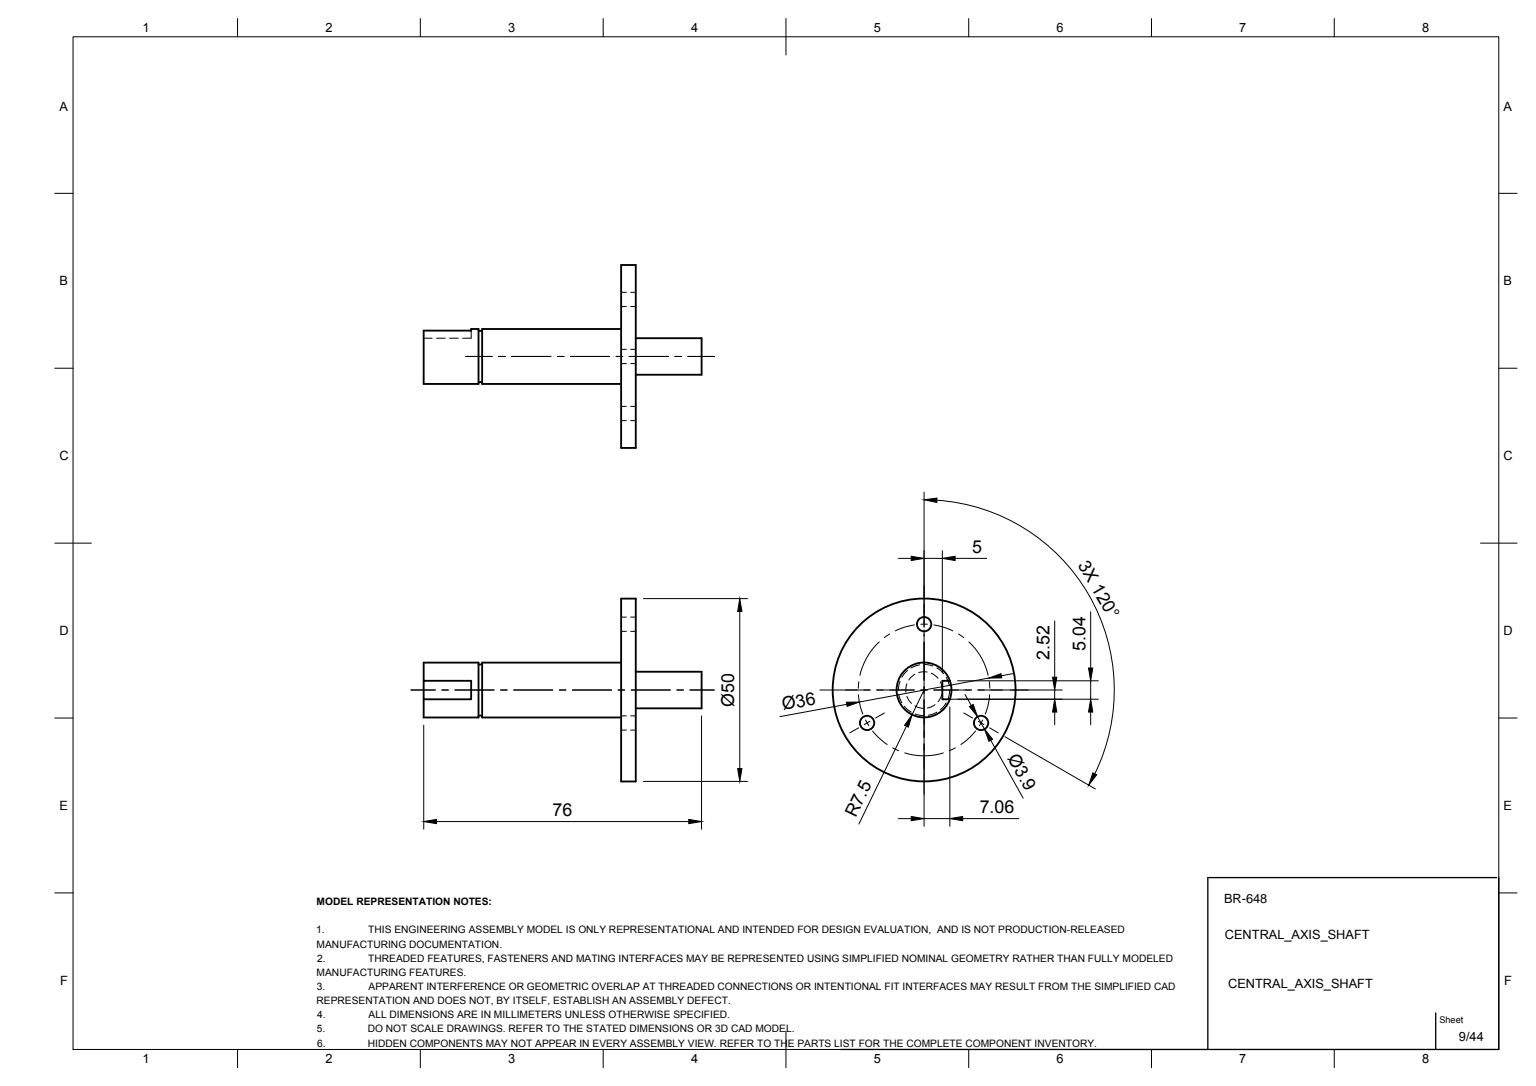
ISO-10303-21;
HEADER;
FILE_DESCRIPTION((''),'2;1');
FILE_NAME('CENTRAL_AXIS_SHAFT.step','2026-10-01T22:05:39-07:00',(''),(''),'','','');
FILE_SCHEMA (('AUTOMOTIVE_DESIGN { 1 0 10303 214 3 1 1 }'));
ENDSEC;
DATA;
#10=MECHANICAL_DESIGN_GEOMETRIC_PRESENTATION_REPRESENTATION('',(#609),#24628);
#525=SHAPE_REPRESENTATION_RELATIONSHIP('SRR','None',#24797,#567) ;
#567=ADVANCED_BREP_SHAPE_REPRESENTATION('',(#651),#24587) ;
#609=STYLED_ITEM('',(#25030),#651) ;
#651=MANIFOLD_SOLID_BREP('CENTRAL_AXIS_SHAFT',#13118) ;
#749=FACE_BOUND('',#3864,.T.) ;
#750=FACE_BOUND('',#3866,.T.) ;
#751=FACE_BOUND('',#3872,.T.) ;
#752=FACE_BOUND('',#3873,.T.) ;
#753=FACE_BOUND('',#3874,.T.) ;
#754=FACE_BOUND('',#3875,.T.) ;
#755=FACE_BOUND('',#3881,.T.) ;
#756=FACE_BOUND('',#3882,.T.) ;
#757=FACE_BOUND('',#3883,.T.) ;
#758=FACE_BOUND('',#3884,.T.) ;
#1071=LINE('',#20189,#1907) ;
#1072=LINE('',#20191,#1908) ;
#1073=LINE('',#20193,#1909) ;
#1074=LINE('',#20194,#1910) ;
#1075=LINE('',#20199,#1911) ;
#1076=LINE('',#20200,#1912) ;
#1077=LINE('',#20204,#1913) ;
#1078=LINE('',#20205,#1914) ;
#1079=LINE('',#20206,#1915) ;
#1080=LINE('',#20208,#1916) ;
#1081=LINE('',#20213,#1917) ;
#1082=LINE('',#20220,#1918) ;
#1083=LINE('',#20229,#1919) ;
#1084=LINE('',#20234,#1920) ;
#1085=LINE('',#20240,#1921) ;
#1086=LINE('',#20246,#1922) ;
#1087=LINE('',#20254,#1923) ;
#1088=LINE('',#20259,#1924) ;
#1907=VECTOR('',#15836,1.) ;
#1908=VECTOR('',#15837,1.) ;
#1909=VECTOR('',#15838,1.) ;
#1910=VECTOR('',#15839,1.) ;
#1911=VECTOR('',#15844,1.) ;
#1912=VECTOR('',#15845,1.) ;
#1913=VECTOR('',#15848,1.) ;
#1914=VECTOR('',#15849,1.) ;
#1915=VECTOR('',#15850,1.) ;
#1916=VECTOR('',#15853,1.) ;
#1917=VECTOR('',#15858,0.75) ;
#1918=VECTOR('',#15867,0.7) ;
#1919=VECTOR('',#15880,0.75) ;
#1920=VECTOR('',#15885,0.195) ;
#1921=VECTOR('',#15892,0.195) ;
#1922=VECTOR('',#15899,0.195) ;
#1923=VECTOR('',#15910,2.5) ;
#1924=VECTOR('',#15915,0.5) ;
#2717=CYLINDRICAL_SURFACE('',#13844,0.75) ;
#2718=CYLINDRICAL_SURFACE('',#13848,0.7) ;
#2719=CYLINDRICAL_SURFACE('',#13854,0.75) ;
#2720=CYLINDRICAL_SURFACE('',#13856,0.195) ;
#2721=CYLINDRICAL_SURFACE('',#13859,0.195) ;
#2722=CYLINDRICAL_SURFACE('',#13862,0.195) ;
#2723=CYLINDRICAL_SURFACE('',#13867,2.5) ;
#2724=CYLINDRICAL_SURFACE('',#13869,0.5) ;
#3027=FACE_OUTER_BOUND('',#3857,.T.) ;
#3028=FACE_OUTER_BOUND('',#3858,.T.) ;
#3029=FACE_OUTER_BOUND('',#3859,.T.) ;
#3030=FACE_OUTER_BOUND('',#3860,.T.) ;
#3031=FACE_OUTER_BOUND('',#3861,.T.) ;
#3032=FACE_OUTER_BOUND('',#3862,.T.) ;
#3033=FACE_OUTER_BOUND('',#3863,.T.) ;
#3034=FACE_OUTER_BOUND('',#3865,.T.) ;
#3035=FACE_OUTER_BOUND('',#3867,.T.) ;
#3036=FACE_OUTER_BOUND('',#3868,.T.) ;
#3037=FACE_OUTER_BOUND('',#3869,.T.) ;
#3038=FACE_OUTER_BOUND('',#3870,.T.) ;
#3039=FACE_OUTER_BOUND('',#3871,.T.) ;
#3040=FACE_OUTER_BOUND('',#3876,.T.) ;
#3041=FACE_OUTER_BOUND('',#3877,.T.) ;
#3042=FACE_OUTER_BOUND('',#3878,.T.) ;
#3043=FACE_OUTER_BOUND('',#3879,.T.) ;
#3044=FACE_OUTER_BOUND('',#3880,.T.) ;
#3857=EDGE_LOOP('',(#8847,#8848,#8849,#8850)) ;
#3858=EDGE_LOOP('',(#8851,#8852,#8853,#8854)) ;
#3859=EDGE_LOOP('',(#8855,#8856,#8857,#8858)) ;
#3860=EDGE_LOOP('',(#8859,#8860,#8861,#8862)) ;
#3861=EDGE_LOOP('',(#8863,#8864,#8865,#8866,#8867,#8868,#8869,#8870)) ;
#3862=EDGE_LOOP('',(#8871,#8872,#8873,#8874)) ;
#3863=EDGE_LOOP('',(#8875)) ;
#3864=EDGE_LOOP('',(#8876)) ;
#3865=EDGE_LOOP('',(#8877)) ;
#3866=EDGE_LOOP('',(#8878)) ;
#3867=EDGE_LOOP('',(#8879,#8880,#8881,#8882)) ;
#3868=EDGE_LOOP('',(#8883,#8884,#8885,#8886)) ;
#3869=EDGE_LOOP('',(#8887,#8888,#8889,#8890)) ;
#3870=EDGE_LOOP('',(#8891,#8892,#8893,#8894)) ;
#3871=EDGE_LOOP('',(#8895)) ;
#3872=EDGE_LOOP('',(#8896)) ;
#3873=EDGE_LOOP('',(#8897)) ;
#3874=EDGE_LOOP('',(#8898)) ;
#3875=EDGE_LOOP('',(#8899)) ;
#3876=EDGE_LOOP('',(#8900,#8901,#8902,#8903)) ;
#3877=EDGE_LOOP('',(#8904,#8905,#8906,#8907)) ;
#3878=EDGE_LOOP('',(#8908)) ;
#3879=EDGE_LOOP('',(#8909,#8910,#8911,#8912,#8913)) ;
#3880=EDGE_LOOP('',(#8914)) ;
#3881=EDGE_LOOP('',(#8915)) ;
#3882=EDGE_LOOP('',(#8916)) ;
#3883=EDGE_LOOP('',(#8917)) ;
#3884=EDGE_LOOP('',(#8918)) ;
#4856=CIRCLE('',#13841,0.75) ;
#4857=CIRCLE('',#13845,0.75) ;
#4858=CIRCLE('',#13846,0.75) ;
#4859=CIRCLE('',#13847,0.75) ;
#4860=CIRCLE('',#13849,0.7) ;
#4861=CIRCLE('',#13850,0.7) ;
#4862=CIRCLE('',#13853,0.75) ;
#4863=CIRCLE('',#13855,0.75) ;
#4864=CIRCLE('',#13857,0.195) ;
#4865=CIRCLE('',#13858,0.195) ;
#4866=CIRCLE('',#13860,0.195) ;
#4867=CIRCLE('',#13861,0.195) ;
#4868=CIRCLE('',#13863,0.195) ;
#4869=CIRCLE('',#13864,0.195) ;
#4870=CIRCLE('',#13866,2.5) ;
#4871=CIRCLE('',#13868,2.5) ;
#4872=CIRCLE('',#13870,0.5) ;
#4873=CIRCLE('',#13871,0.5) ;
#5657=VERTEX_POINT('',#20187) ;
#5658=VERTEX_POINT('',#20188) ;
#5659=VERTEX_POINT('',#20190) ;
#5660=VERTEX_POINT('',#20192) ;
#5661=VERTEX_POINT('',#20196) ;
#5662=VERTEX_POINT('',#20198) ;
#5663=VERTEX_POINT('',#20202) ;
#5664=VERTEX_POINT('',#20203) ;
#5665=VERTEX_POINT('',#20210) ;
#5666=VERTEX_POINT('',#20212) ;
#5667=VERTEX_POINT('',#20217) ;
#5668=VERTEX_POINT('',#20219) ;
#5669=VERTEX_POINT('',#20224) ;
#5670=VERTEX_POINT('',#20227) ;
#5671=VERTEX_POINT('',#20231) ;
#5672=VERTEX_POINT('',#20233) ;
#5673=VERTEX_POINT('',#20237) ;
#5674=VERTEX_POINT('',#20239) ;
#5675=VERTEX_POINT('',#20243) ;
#5676=VERTEX_POINT('',#20245) ;
#5677=VERTEX_POINT('',#20249) ;
#5678=VERTEX_POINT('',#20252) ;
#5679=VERTEX_POINT('',#20256) ;
#5680=VERTEX_POINT('',#20258) ;
#6913=EDGE_CURVE('',#5657,#5658,#1071,.T.) ;
#6914=EDGE_CURVE('',#5659,#5657,#1072,.T.) ;
#6915=EDGE_CURVE('',#5660,#5659,#1073,.T.) ;
#6916=EDGE_CURVE('',#5658,#5660,#1074,.T.) ;
#6917=EDGE_CURVE('',#5660,#5661,#4856,.T.) ;
#6918=EDGE_CURVE('',#5659,#5662,#1075,.T.) ;
#6919=EDGE_CURVE('',#5662,#5661,#1076,.T.) ;
#6920=EDGE_CURVE('',#5663,#5664,#1077,.T.) ;
#6921=EDGE_CURVE('',#5661,#5663,#1078,.T.) ;
#6922=EDGE_CURVE('',#5664,#5662,#1079,.T.) ;
#6923=EDGE_CURVE('',#5664,#5657,#1080,.T.) ;
#6924=EDGE_CURVE('',#5665,#5665,#4857,.T.) ;
#6925=EDGE_CURVE('',#5665,#5666,#1081,.T.) ;
#6926=EDGE_CURVE('',#5658,#5666,#4858,.T.) ;
#6927=EDGE_CURVE('',#5666,#5663,#4859,.T.) ;
#6928=EDGE_CURVE('',#5667,#5667,#4860,.T.) ;
#6929=EDGE_CURVE('',#5667,#5668,#1082,.T.) ;
#6930=EDGE_CURVE('',#5668,#5668,#4861,.T.) ;
#6931=EDGE_CURVE('',#5669,#5669,#4862,.T.) ;
#6932=EDGE_CURVE('',#5670,#5670,#4863,.T.) ;
#6933=EDGE_CURVE('',#5670,#5669,#1083,.T.) ;
#6934=EDGE_CURVE('',#5671,#5671,#4864,.T.) ;
#6935=EDGE_CURVE('',#5671,#5672,#1084,.T.) ;
#6936=EDGE_CURVE('',#5672,#5672,#4865,.T.) ;
#6937=EDGE_CURVE('',#5673,#5673,#4866,.T.) ;
#6938=EDGE_CURVE('',#5673,#5674,#1085,.T.) ;
#6939=EDGE_CURVE('',#5674,#5674,#4867,.T.) ;
#6940=EDGE_CURVE('',#5675,#5675,#4868,.T.) ;
#6941=EDGE_CURVE('',#5675,#5676,#1086,.T.) ;
#6942=EDGE_CURVE('',#5676,#5676,#4869,.T.) ;
#6943=EDGE_CURVE('',#5677,#5677,#4870,.T.) ;
#6944=EDGE_CURVE('',#5678,#5678,#4871,.T.) ;
#6945=EDGE_CURVE('',#5678,#5677,#1087,.T.) ;
#6946=EDGE_CURVE('',#5679,#5679,#4872,.T.) ;
#6947=EDGE_CURVE('',#5679,#5680,#1088,.T.) ;
#6948=EDGE_CURVE('',#5680,#5680,#4873,.T.) ;
#8847=ORIENTED_EDGE('',*,*,#6913,.F.) ;
#8848=ORIENTED_EDGE('',*,*,#6914,.F.) ;
#8849=ORIENTED_EDGE('',*,*,#6915,.F.) ;
#8850=ORIENTED_EDGE('',*,*,#6916,.F.) ;
#8851=ORIENTED_EDGE('',*,*,#6917,.F.) ;
#8852=ORIENTED_EDGE('',*,*,#6915,.T.) ;
#8853=ORIENTED_EDGE('',*,*,#6918,.T.) ;
#8854=ORIENTED_EDGE('',*,*,#6919,.T.) ;
#8855=ORIENTED_EDGE('',*,*,#6920,.F.) ;
#8856=ORIENTED_EDGE('',*,*,#6921,.F.) ;
#8857=ORIENTED_EDGE('',*,*,#6919,.F.) ;
#8858=ORIENTED_EDGE('',*,*,#6922,.F.) ;
#8859=ORIENTED_EDGE('',*,*,#6923,.F.) ;
#8860=ORIENTED_EDGE('',*,*,#6922,.T.) ;
#8861=ORIENTED_EDGE('',*,*,#6918,.F.) ;
#8862=ORIENTED_EDGE('',*,*,#6914,.T.) ;
#8863=ORIENTED_EDGE('',*,*,#6924,.T.) ;
#8864=ORIENTED_EDGE('',*,*,#6925,.T.) ;
#8865=ORIENTED_EDGE('',*,*,#6926,.F.) ;
#8866=ORIENTED_EDGE('',*,*,#6916,.T.) ;
#8867=ORIENTED_EDGE('',*,*,#6917,.T.) ;
#8868=ORIENTED_EDGE('',*,*,#6921,.T.) ;
#8869=ORIENTED_EDGE('',*,*,#6927,.F.) ;
#8870=ORIENTED_EDGE('',*,*,#6925,.F.) ;
#8871=ORIENTED_EDGE('',*,*,#6928,.T.) ;
#8872=ORIENTED_EDGE('',*,*,#6929,.T.) ;
#8873=ORIENTED_EDGE('',*,*,#6930,.T.) ;
#8874=ORIENTED_EDGE('',*,*,#6929,.F.) ;
#8875=ORIENTED_EDGE('',*,*,#6924,.F.) ;
#8876=ORIENTED_EDGE('',*,*,#6930,.F.) ;
#8877=ORIENTED_EDGE('',*,*,#6931,.F.) ;
#8878=ORIENTED_EDGE('',*,*,#6928,.F.) ;
#8879=ORIENTED_EDGE('',*,*,#6932,.T.) ;
#8880=ORIENTED_EDGE('',*,*,#6933,.T.) ;
#8881=ORIENTED_EDGE('',*,*,#6931,.T.) ;
#8882=ORIENTED_EDGE('',*,*,#6933,.F.) ;
#8883=ORIENTED_EDGE('',*,*,#6934,.F.) ;
#8884=ORIENTED_EDGE('',*,*,#6935,.T.) ;
#8885=ORIENTED_EDGE('',*,*,#6936,.F.) ;
#8886=ORIENTED_EDGE('',*,*,#6935,.F.) ;
#8887=ORIENTED_EDGE('',*,*,#6937,.F.) ;
#8888=ORIENTED_EDGE('',*,*,#6938,.T.) ;
#8889=ORIENTED_EDGE('',*,*,#6939,.F.) ;
#8890=ORIENTED_EDGE('',*,*,#6938,.F.) ;
#8891=ORIENTED_EDGE('',*,*,#6940,.F.) ;
#8892=ORIENTED_EDGE('',*,*,#6941,.T.) ;
#8893=ORIENTED_EDGE('',*,*,#6942,.F.) ;
#8894=ORIENTED_EDGE('',*,*,#6941,.F.) ;
#8895=ORIENTED_EDGE('',*,*,#6943,.T.) ;
#8896=ORIENTED_EDGE('',*,*,#6934,.T.) ;
#8897=ORIENTED_EDGE('',*,*,#6937,.T.) ;
#8898=ORIENTED_EDGE('',*,*,#6940,.T.) ;
#8899=ORIENTED_EDGE('',*,*,#6932,.F.) ;
#8900=ORIENTED_EDGE('',*,*,#6944,.F.) ;
#8901=ORIENTED_EDGE('',*,*,#6945,.T.) ;
#8902=ORIENTED_EDGE('',*,*,#6943,.F.) ;
#8903=ORIENTED_EDGE('',*,*,#6945,.F.) ;
#8904=ORIENTED_EDGE('',*,*,#6946,.F.) ;
#8905=ORIENTED_EDGE('',*,*,#6947,.T.) ;
#8906=ORIENTED_EDGE('',*,*,#6948,.F.) ;
#8907=ORIENTED_EDGE('',*,*,#6947,.F.) ;
#8908=ORIENTED_EDGE('',*,*,#6946,.T.) ;
#8909=ORIENTED_EDGE('',*,*,#6913,.T.) ;
#8910=ORIENTED_EDGE('',*,*,#6926,.T.) ;
#8911=ORIENTED_EDGE('',*,*,#6927,.T.) ;
#8912=ORIENTED_EDGE('',*,*,#6920,.T.) ;
#8913=ORIENTED_EDGE('',*,*,#6923,.T.) ;
#8914=ORIENTED_EDGE('',*,*,#6944,.T.) ;
#8915=ORIENTED_EDGE('',*,*,#6936,.T.) ;
#8916=ORIENTED_EDGE('',*,*,#6939,.T.) ;
#8917=ORIENTED_EDGE('',*,*,#6942,.T.) ;
#8918=ORIENTED_EDGE('',*,*,#6948,.T.) ;
#12026=PLANE('',#13839) ;
#12027=PLANE('',#13840) ;
#12028=PLANE('',#13842) ;
#12029=PLANE('',#13843) ;
#12030=PLANE('',#13851) ;
#12031=PLANE('',#13852) ;
#12032=PLANE('',#13865) ;
#12033=PLANE('',#13872) ;
#12034=PLANE('',#13873) ;
#12035=PLANE('',#13874) ;
#12422=ADVANCED_FACE('',(#3027),#12026,.F.) ;
#12423=ADVANCED_FACE('',(#3028),#12027,.T.) ;
#12424=ADVANCED_FACE('',(#3029),#12028,.T.) ;
#12425=ADVANCED_FACE('',(#3030),#12029,.T.) ;
#12426=ADVANCED_FACE('',(#3031),#2717,.T.) ;
#12427=ADVANCED_FACE('',(#3032),#2718,.T.) ;
#12428=ADVANCED_FACE('',(#3033,#749),#12030,.F.) ;
#12429=ADVANCED_FACE('',(#3034,#750),#12031,.F.) ;
#12430=ADVANCED_FACE('',(#3035),#2719,.T.) ;
#12431=ADVANCED_FACE('',(#3036),#2720,.F.) ;
#12432=ADVANCED_FACE('',(#3037),#2721,.F.) ;
#12433=ADVANCED_FACE('',(#3038),#2722,.F.) ;
#12434=ADVANCED_FACE('',(#3039,#751,#752,#753,#754),#12032,.T.) ;
#12435=ADVANCED_FACE('',(#3040),#2723,.T.) ;
#12436=ADVANCED_FACE('',(#3041),#2724,.T.) ;
#12437=ADVANCED_FACE('',(#3042),#12033,.T.) ;
#12438=ADVANCED_FACE('',(#3043),#12034,.T.) ;
#12439=ADVANCED_FACE('',(#3044,#755,#756,#757,#758),#12035,.T.) ;
#13118=CLOSED_SHELL('',(#12422,#12423,#12424,#12425,#12426,#12427,#12428,
#12429,#12430,#12431,#12432,#12433,#12434,#12435,#12436,#12437,#12438,#12439)) ;
#13838=AXIS2_PLACEMENT_3D('',#20185,#15832,#15833) ;
#13839=AXIS2_PLACEMENT_3D('',#20186,#15834,#15835) ;
#13840=AXIS2_PLACEMENT_3D('',#20195,#15840,#15841) ;
#13841=AXIS2_PLACEMENT_3D('',#20197,#15842,#15843) ;
#13842=AXIS2_PLACEMENT_3D('',#20201,#15846,#15847) ;
#13843=AXIS2_PLACEMENT_3D('',#20207,#15851,#15852) ;
#13844=AXIS2_PLACEMENT_3D('',#20209,#15854,#15855) ;
#13845=AXIS2_PLACEMENT_3D('',#20211,#15856,#15857) ;
#13846=AXIS2_PLACEMENT_3D('',#20214,#15859,#15860) ;
#13847=AXIS2_PLACEMENT_3D('',#20215,#15861,#15862) ;
#13848=AXIS2_PLACEMENT_3D('',#20216,#15863,#15864) ;
#13849=AXIS2_PLACEMENT_3D('',#20218,#15865,#15866) ;
#13850=AXIS2_PLACEMENT_3D('',#20221,#15868,#15869) ;
#13851=AXIS2_PLACEMENT_3D('',#20222,#15870,#15871) ;
#13852=AXIS2_PLACEMENT_3D('',#20223,#15872,#15873) ;
#13853=AXIS2_PLACEMENT_3D('',#20225,#15874,#15875) ;
#13854=AXIS2_PLACEMENT_3D('',#20226,#15876,#15877) ;
#13855=AXIS2_PLACEMENT_3D('',#20228,#15878,#15879) ;
#13856=AXIS2_PLACEMENT_3D('',#20230,#15881,#15882) ;
#13857=AXIS2_PLACEMENT_3D('',#20232,#15883,#15884) ;
#13858=AXIS2_PLACEMENT_3D('',#20235,#15886,#15887) ;
#13859=AXIS2_PLACEMENT_3D('',#20236,#15888,#15889) ;
#13860=AXIS2_PLACEMENT_3D('',#20238,#15890,#15891) ;
#13861=AXIS2_PLACEMENT_3D('',#20241,#15893,#15894) ;
#13862=AXIS2_PLACEMENT_3D('',#20242,#15895,#15896) ;
#13863=AXIS2_PLACEMENT_3D('',#20244,#15897,#15898) ;
#13864=AXIS2_PLACEMENT_3D('',#20247,#15900,#15901) ;
#13865=AXIS2_PLACEMENT_3D('',#20248,#15902,#15903) ;
#13866=AXIS2_PLACEMENT_3D('',#20250,#15904,#15905) ;
#13867=AXIS2_PLACEMENT_3D('',#20251,#15906,#15907) ;
#13868=AXIS2_PLACEMENT_3D('',#20253,#15908,#15909) ;
#13869=AXIS2_PLACEMENT_3D('',#20255,#15911,#15912) ;
#13870=AXIS2_PLACEMENT_3D('',#20257,#15913,#15914) ;
#13871=AXIS2_PLACEMENT_3D('',#20260,#15916,#15917) ;
#13872=AXIS2_PLACEMENT_3D('',#20261,#15918,#15919) ;
#13873=AXIS2_PLACEMENT_3D('',#20262,#15920,#15921) ;
#13874=AXIS2_PLACEMENT_3D('',#20263,#15922,#15923) ;
#15832=DIRECTION('axis',(0.,0.,1.)) ;
#15833=DIRECTION('refdir',(1.,0.,0.)) ;
#15834=DIRECTION('center_axis',(0.,0.,1.)) ;
#15835=DIRECTION('ref_axis',(1.,0.,0.)) ;
#15836=DIRECTION('',(1.,0.,0.)) ;
#15837=DIRECTION('',(0.,-1.,0.)) ;
#15838=DIRECTION('',(-1.,0.,0.)) ;
#15839=DIRECTION('',(0.,1.,0.)) ;
#15840=DIRECTION('center_axis',(0.,-1.,0.)) ;
#15841=DIRECTION('ref_axis',(0.,0.,-1.)) ;
#15842=DIRECTION('center_axis',(0.,1.,0.)) ;
#15843=DIRECTION('ref_axis',(1.,0.,0.)) ;
#15844=DIRECTION('',(0.,0.,-1.)) ;
#15845=DIRECTION('',(1.,0.,0.)) ;
#15846=DIRECTION('center_axis',(0.,0.,1.)) ;
#15847=DIRECTION('ref_axis',(1.,0.,0.)) ;
#15848=DIRECTION('',(-1.,0.,0.)) ;
#15849=DIRECTION('',(0.,-1.,0.)) ;
#15850=DIRECTION('',(0.,1.,0.)) ;
#15851=DIRECTION('center_axis',(1.,0.,0.)) ;
#15852=DIRECTION('ref_axis',(0.,0.,-1.)) ;
#15853=DIRECTION('',(0.,0.,1.)) ;
#15854=DIRECTION('center_axis',(0.,1.,0.)) ;
#15855=DIRECTION('ref_axis',(1.,0.,0.)) ;
#15856=DIRECTION('center_axis',(0.,-1.,0.)) ;
#15857=DIRECTION('ref_axis',(1.,0.,0.)) ;
#15858=DIRECTION('',(0.,-1.,0.)) ;
#15859=DIRECTION('center_axis',(0.,-1.,0.)) ;
#15860=DIRECTION('ref_axis',(1.,0.,0.)) ;
#15861=DIRECTION('center_axis',(0.,-1.,0.)) ;
#15862=DIRECTION('ref_axis',(1.,0.,0.)) ;
#15863=DIRECTION('center_axis',(0.,1.,0.)) ;
#15864=DIRECTION('ref_axis',(1.,0.,0.)) ;
#15865=DIRECTION('center_axis',(0.,-1.,0.)) ;
#15866=DIRECTION('ref_axis',(1.,0.,0.)) ;
#15867=DIRECTION('',(0.,-1.,0.)) ;
#15868=DIRECTION('center_axis',(0.,1.,0.)) ;
#15869=DIRECTION('ref_axis',(1.,0.,0.)) ;
#15870=DIRECTION('center_axis',(0.,-1.,0.)) ;
#15871=DIRECTION('ref_axis',(-1.,0.,0.)) ;
#15872=DIRECTION('center_axis',(0.,1.,0.)) ;
#15873=DIRECTION('ref_axis',(1.,0.,0.)) ;
#15874=DIRECTION('center_axis',(0.,1.,0.)) ;
#15875=DIRECTION('ref_axis',(1.,0.,0.)) ;
#15876=DIRECTION('center_axis',(0.,1.,0.)) ;
#15877=DIRECTION('ref_axis',(1.,0.,0.)) ;
#15878=DIRECTION('center_axis',(0.,-1.,0.)) ;
#15879=DIRECTION('ref_axis',(1.,0.,0.)) ;
#15880=DIRECTION('',(0.,-1.,0.)) ;
#15881=DIRECTION('center_axis',(0.,1.,0.)) ;
#15882=DIRECTION('ref_axis',(1.,0.,0.)) ;
#15883=DIRECTION('center_axis',(0.,1.,0.)) ;
#15884=DIRECTION('ref_axis',(1.,0.,0.)) ;
#15885=DIRECTION('',(0.,1.,0.)) ;
#15886=DIRECTION('center_axis',(0.,-1.,0.)) ;
#15887=DIRECTION('ref_axis',(1.,0.,0.)) ;
#15888=DIRECTION('center_axis',(0.,1.,0.)) ;
#15889=DIRECTION('ref_axis',(1.,0.,0.)) ;
#15890=DIRECTION('center_axis',(0.,1.,0.)) ;
#15891=DIRECTION('ref_axis',(1.,0.,0.)) ;
#15892=DIRECTION('',(0.,1.,0.)) ;
#15893=DIRECTION('center_axis',(0.,-1.,0.)) ;
#15894=DIRECTION('ref_axis',(1.,0.,0.)) ;
#15895=DIRECTION('center_axis',(0.,1.,0.)) ;
#15896=DIRECTION('ref_axis',(1.,0.,0.)) ;
#15897=DIRECTION('center_axis',(0.,1.,0.)) ;
#15898=DIRECTION('ref_axis',(1.,0.,0.)) ;
#15899=DIRECTION('',(0.,1.,0.)) ;
#15900=DIRECTION('center_axis',(0.,-1.,0.)) ;
#15901=DIRECTION('ref_axis',(1.,0.,0.)) ;
#15902=DIRECTION('center_axis',(0.,-1.,0.)) ;
#15903=DIRECTION('ref_axis',(-1.,0.,0.)) ;
#15904=DIRECTION('center_axis',(0.,-1.,0.)) ;
#15905=DIRECTION('ref_axis',(1.,0.,0.)) ;
#15906=DIRECTION('center_axis',(0.,1.,0.)) ;
#15907=DIRECTION('ref_axis',(1.,0.,0.)) ;
#15908=DIRECTION('center_axis',(0.,1.,0.)) ;
#15909=DIRECTION('ref_axis',(1.,0.,0.)) ;
#15910=DIRECTION('',(0.,-1.,0.)) ;
#15911=DIRECTION('center_axis',(0.,1.,0.)) ;
#15912=DIRECTION('ref_axis',(1.,0.,0.)) ;
#15913=DIRECTION('center_axis',(0.,1.,0.)) ;
#15914=DIRECTION('ref_axis',(1.,0.,0.)) ;
#15915=DIRECTION('',(0.,-1.,0.)) ;
#15916=DIRECTION('center_axis',(0.,-1.,0.)) ;
#15917=DIRECTION('ref_axis',(1.,0.,0.)) ;
#15918=DIRECTION('center_axis',(0.,1.,0.)) ;
#15919=DIRECTION('ref_axis',(1.,0.,0.)) ;
#15920=DIRECTION('center_axis',(0.,-1.,0.)) ;
#15921=DIRECTION('ref_axis',(-1.,0.,0.)) ;
#15922=DIRECTION('center_axis',(0.,1.,0.)) ;
#15923=DIRECTION('ref_axis',(1.,0.,0.)) ;
#20185=CARTESIAN_POINT('',(0.,0.,0.)) ;
#20186=CARTESIAN_POINT('Origin',(0.65,-6.2,0.252)) ;
#20187=CARTESIAN_POINT('',(0.5,-6.8,0.252)) ;
#20188=CARTESIAN_POINT('',(0.706396489232499,-6.8,0.252)) ;
#20189=CARTESIAN_POINT('',(0.325,-6.8,0.252)) ;
#20190=CARTESIAN_POINT('',(0.5,-5.5,0.252)) ;
#20191=CARTESIAN_POINT('',(0.5,-6.2,0.252)) ;
#20192=CARTESIAN_POINT('',(0.706396489232499,-5.5,0.252)) ;
#20193=CARTESIAN_POINT('',(0.65,-5.5,0.252)) ;
#20194=CARTESIAN_POINT('',(0.706396489232499,-3.9,0.252)) ;
#20195=CARTESIAN_POINT('Origin',(0.65,-5.5,0.)) ;
#20196=CARTESIAN_POINT('',(0.706396489232499,-5.5,-0.252)) ;
#20197=CARTESIAN_POINT('Origin',(0.,-5.5,0.)) ;
#20198=CARTESIAN_POINT('',(0.5,-5.5,-0.252)) ;
#20199=CARTESIAN_POINT('',(0.5,-5.5,0.)) ;
#20200=CARTESIAN_POINT('',(0.65,-5.5,-0.252)) ;
#20201=CARTESIAN_POINT('Origin',(0.65,-6.2,-0.252)) ;
#20202=CARTESIAN_POINT('',(0.706396489232499,-6.8,-0.252)) ;
#20203=CARTESIAN_POINT('',(0.5,-6.8,-0.252)) ;
#20204=CARTESIAN_POINT('',(0.325,-6.8,-0.252)) ;
#20205=CARTESIAN_POINT('',(0.706396489232499,-3.9,-0.252)) ;
#20206=CARTESIAN_POINT('',(0.5,-6.2,-0.252)) ;
#20207=CARTESIAN_POINT('Origin',(0.5,-6.2,0.)) ;
#20208=CARTESIAN_POINT('',(0.5,-6.8,0.)) ;
#20209=CARTESIAN_POINT('Origin',(0.,-3.9,0.)) ;
#20210=CARTESIAN_POINT('',(-0.75,-5.3,-9.18485099360515E-17)) ;
#20211=CARTESIAN_POINT('Origin',(0.,-5.3,0.)) ;
#20212=CARTESIAN_POINT('',(-0.75,-6.8,9.18485099360515E-17)) ;
#20213=CARTESIAN_POINT('',(-0.75,-3.9,9.18485099360515E-17)) ;
#20214=CARTESIAN_POINT('Origin',(0.,-6.8,0.)) ;
#20215=CARTESIAN_POINT('Origin',(0.,-6.8,0.)) ;
#20216=CARTESIAN_POINT('Origin',(0.,-5.25,0.)) ;
#20217=CARTESIAN_POINT('',(-0.7,-5.2,-8.57252759403147E-17)) ;
#20218=CARTESIAN_POINT('Origin',(0.,-5.2,0.)) ;
#20219=CARTESIAN_POINT('',(-0.7,-5.3,8.57252759403147E-17)) ;
#20220=CARTESIAN_POINT('',(-0.7,-5.25,8.57252759403147E-17)) ;
#20221=CARTESIAN_POINT('Origin',(0.,-5.3,0.)) ;
#20222=CARTESIAN_POINT('Origin',(0.,-5.3,0.)) ;
#20223=CARTESIAN_POINT('Origin',(0.,-5.2,0.)) ;
#20224=CARTESIAN_POINT('',(-0.75,-5.2,9.18485099360515E-17)) ;
#20225=CARTESIAN_POINT('Origin',(0.,-5.2,0.)) ;
#20226=CARTESIAN_POINT('Origin',(0.,-3.9,0.)) ;
#20227=CARTESIAN_POINT('',(-0.75,-1.4,-9.18485099360515E-17)) ;
#20228=CARTESIAN_POINT('Origin',(0.,-1.4,0.)) ;
#20229=CARTESIAN_POINT('',(-0.75,-3.9,9.18485099360515E-17)) ;
#20230=CARTESIAN_POINT('Origin',(1.55884572681199,-1.2,-0.900000000000001)) ;
#20231=CARTESIAN_POINT('',(1.36384572681199,-1.4,-0.900000000000001)) ;
#20232=CARTESIAN_POINT('Origin',(1.55884572681199,-1.4,-0.900000000000001)) ;
#20233=CARTESIAN_POINT('',(1.36384572681199,-1.,-0.900000000000001)) ;
#20234=CARTESIAN_POINT('',(1.36384572681199,-1.2,-0.900000000000001)) ;
#20235=CARTESIAN_POINT('Origin',(1.55884572681199,-1.,-0.900000000000001)) ;
#20236=CARTESIAN_POINT('Origin',(-1.55884572681199,-1.2,-0.9)) ;
#20237=CARTESIAN_POINT('',(-1.75384572681199,-1.4,-0.9)) ;
#20238=CARTESIAN_POINT('Origin',(-1.55884572681199,-1.4,-0.9)) ;
#20239=CARTESIAN_POINT('',(-1.75384572681199,-1.,-0.9)) ;
#20240=CARTESIAN_POINT('',(-1.75384572681199,-1.2,-0.9)) ;
#20241=CARTESIAN_POINT('Origin',(-1.55884572681199,-1.,-0.9)) ;
#20242=CARTESIAN_POINT('Origin',(1.10218211923262E-16,-1.2,1.8)) ;
#20243=CARTESIAN_POINT('',(-0.195,-1.4,1.8)) ;
#20244=CARTESIAN_POINT('Origin',(1.10218211923262E-16,-1.4,1.8)) ;
#20245=CARTESIAN_POINT('',(-0.195,-1.,1.8)) ;
#20246=CARTESIAN_POINT('',(-0.195,-1.2,1.8)) ;
#20247=CARTESIAN_POINT('Origin',(1.10218211923262E-16,-1.,1.8)) ;
#20248=CARTESIAN_POINT('Origin',(0.,-1.4,0.)) ;
#20249=CARTESIAN_POINT('',(-2.5,-1.4,3.06161699786838E-16)) ;
#20250=CARTESIAN_POINT('Origin',(0.,-1.4,0.)) ;
#20251=CARTESIAN_POINT('Origin',(0.,-1.2,0.)) ;
#20252=CARTESIAN_POINT('',(-2.5,-1.,3.06161699786838E-16)) ;
#20253=CARTESIAN_POINT('Origin',(0.,-1.,0.)) ;
#20254=CARTESIAN_POINT('',(-2.5,-1.2,3.06161699786838E-16)) ;
#20255=CARTESIAN_POINT('Origin',(0.,-0.1,0.)) ;
#20256=CARTESIAN_POINT('',(-0.5,0.8,6.12323399573677E-17)) ;
#20257=CARTESIAN_POINT('Origin',(0.,0.8,0.)) ;
#20258=CARTESIAN_POINT('',(-0.5,-1.,6.12323399573677E-17)) ;
#20259=CARTESIAN_POINT('',(-0.5,-0.1,6.12323399573677E-17)) ;
#20260=CARTESIAN_POINT('Origin',(0.,-1.,0.)) ;
#20261=CARTESIAN_POINT('Origin',(0.,0.8,0.)) ;
#20262=CARTESIAN_POINT('Origin',(0.,-6.8,0.)) ;
#20263=CARTESIAN_POINT('Origin',(0.,-1.,0.)) ;
#24539=UNCERTAINTY_MEASURE_WITH_UNIT(LENGTH_MEASURE(0.001),#24629,
'DISTANCE_ACCURACY_VALUE',
'Maximum model space distance between geometric entities at asserted c
onnectivities') ;
#24580=UNCERTAINTY_MEASURE_WITH_UNIT(LENGTH_MEASURE(0.001),#24629,
'DISTANCE_ACCURACY_VALUE',
'Maximum model space distance between geometric entities at asserted c
onnectivities') ;
#24587=(
GEOMETRIC_REPRESENTATION_CONTEXT(3)
GLOBAL_UNCERTAINTY_ASSIGNED_CONTEXT((#24539))
GLOBAL_UNIT_ASSIGNED_CONTEXT((#24629,#24631,#24632))
REPRESENTATION_CONTEXT('','3D')
) ;
#24628=(
GEOMETRIC_REPRESENTATION_CONTEXT(3)
GLOBAL_UNCERTAINTY_ASSIGNED_CONTEXT((#24580))
GLOBAL_UNIT_ASSIGNED_CONTEXT((#24629,#24631,#24632))
REPRESENTATION_CONTEXT('','3D')
) ;
#24629=(
LENGTH_UNIT()
NAMED_UNIT(*)
SI_UNIT(.CENTI.,.METRE.)
) ;
#24631=(
NAMED_UNIT(*)
PLANE_ANGLE_UNIT()
SI_UNIT($,.RADIAN.)
) ;
#24632=(
NAMED_UNIT(*)
SI_UNIT($,.STERADIAN.)
SOLID_ANGLE_UNIT()
) ;
#24639=SHAPE_DEFINITION_REPRESENTATION(#24686,#24797) ;
#24686=PRODUCT_DEFINITION_SHAPE('',$,#24845) ;
#24797=SHAPE_REPRESENTATION('',(#13838),#24587) ;
#24838=PRODUCT_DEFINITION_CONTEXT('part definition',#24981,'design') ;
#24845=PRODUCT_DEFINITION('CENTRAL_AXIS_SHAFT',
'CENTRAL_AXIS_SHAFT',#24892,#24838) ;
#24892=PRODUCT_DEFINITION_FORMATION('',$,#24989) ;
#24981=APPLICATION_CONTEXT(
'Core Data for Automotive Mechanical Design Process') ;
#24982=PRODUCT_CONTEXT('part definition',#24981,'mechanical') ;
#24989=PRODUCT('CENTRAL_AXIS_SHAFT','CENTRAL_AXIS_SHAFT',$,(#24982)) ;
#25030=PRESENTATION_STYLE_ASSIGNMENT((#25040)) ;
#25040=SURFACE_STYLE_USAGE(.BOTH.,#25050) ;
#25050=SURFACE_SIDE_STYLE('',(#25060)) ;
#25060=SURFACE_STYLE_FILL_AREA(#25070) ;
#25070=FILL_AREA_STYLE('Steel - Satin',(#25080)) ;
#25080=FILL_AREA_STYLE_COLOUR('Steel - Satin',#25090) ;
#25090=COLOUR_RGB('Steel - Satin', 0.66274510, 0.83137255, 0.94901961) ;
ENDSEC;
END-ISO-10303-21;
